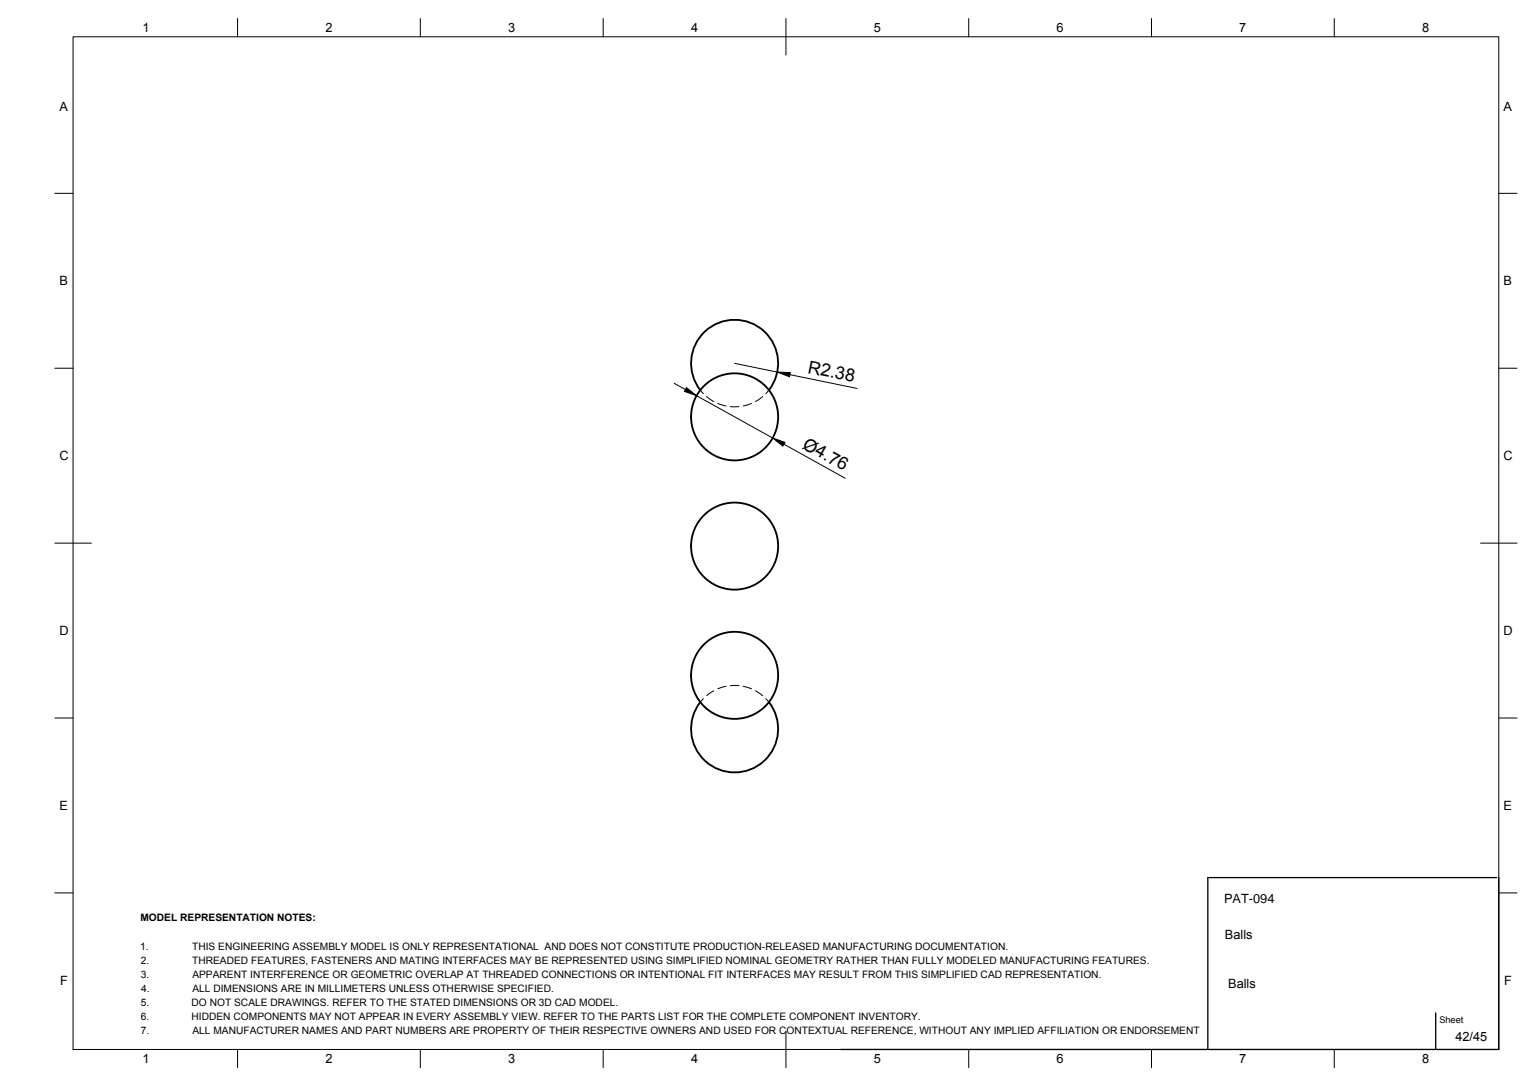
ISO-10303-21;
HEADER;
/* Generated by software containing ST-Developer
 * from STEP Tools, Inc. (www.steptools.com) 
 */

FILE_DESCRIPTION(
/* description */ ('Shaft runout checking stand'),
/* implementation_level */ '2;1');

FILE_NAME(
/* name */ 'Balls.step',
/* time_stamp */ '2026-11-02T21:12:33-08:00',
/* author */ (''),
/* organization */ (''),
/* preprocessor_version */ 'ST-DEVELOPER v20.2',
/* originating_system */ 'Autodesk Translation Framework v15.17.0.0',
/* authorisation */ '');

FILE_SCHEMA (('AUTOMOTIVE_DESIGN { 1 0 10303 214 3 1 1 }'));
ENDSEC;

DATA;
#10=MECHANICAL_DESIGN_GEOMETRIC_PRESENTATION_REPRESENTATION('',(#500,#501,#502,#503,#504,#505,#506,#507),#11748);
#11=SPHERICAL_SURFACE('',#7363,0.23815);
#12=SPHERICAL_SURFACE('',#7365,0.23815);
#13=SPHERICAL_SURFACE('',#7367,0.23815);
#14=SPHERICAL_SURFACE('',#7369,0.23815);
#15=SPHERICAL_SURFACE('',#7371,0.23815);
#16=SPHERICAL_SURFACE('',#7373,0.23815);
#17=SPHERICAL_SURFACE('',#7375,0.23815);
#18=SPHERICAL_SURFACE('',#7377,0.23815);
#414=SHAPE_REPRESENTATION_RELATIONSHIP('SRR','None',#11966,#457);
#457=ADVANCED_BREP_SHAPE_REPRESENTATION('',(#548,#549,#550,#551,#552,#553,
#554,#555),#11742);
#500=STYLED_ITEM('',(#12170),#548);
#501=STYLED_ITEM('',(#12170),#549);
#502=STYLED_ITEM('',(#12170),#550);
#503=STYLED_ITEM('',(#12170),#551);
#504=STYLED_ITEM('',(#12170),#552);
#505=STYLED_ITEM('',(#12170),#553);
#506=STYLED_ITEM('',(#12170),#554);
#507=STYLED_ITEM('',(#12170),#555);
#548=MANIFOLD_SOLID_BREP('Body1',#6246);
#549=MANIFOLD_SOLID_BREP('Body2',#6247);
#550=MANIFOLD_SOLID_BREP('Body3',#6248);
#551=MANIFOLD_SOLID_BREP('Body4',#6249);
#552=MANIFOLD_SOLID_BREP('Body5',#6250);
#553=MANIFOLD_SOLID_BREP('Body6',#6251);
#554=MANIFOLD_SOLID_BREP('Body7',#6252);
#555=MANIFOLD_SOLID_BREP('Body8',#6253);
#876=CIRCLE('',#7364,0.23815);
#877=CIRCLE('',#7366,0.23815);
#878=CIRCLE('',#7368,0.23815);
#879=CIRCLE('',#7370,0.23815);
#880=CIRCLE('',#7372,0.23815);
#881=CIRCLE('',#7374,0.23815);
#882=CIRCLE('',#7376,0.23815);
#883=CIRCLE('',#7378,0.23815);
#1359=FACE_OUTER_BOUND('',#1827,.T.);
#1360=FACE_OUTER_BOUND('',#1828,.T.);
#1361=FACE_OUTER_BOUND('',#1829,.T.);
#1362=FACE_OUTER_BOUND('',#1830,.T.);
#1363=FACE_OUTER_BOUND('',#1831,.T.);
#1364=FACE_OUTER_BOUND('',#1832,.T.);
#1365=FACE_OUTER_BOUND('',#1833,.T.);
#1366=FACE_OUTER_BOUND('',#1834,.T.);
#1827=EDGE_LOOP('',(#5420,#5421));
#1828=EDGE_LOOP('',(#5422,#5423));
#1829=EDGE_LOOP('',(#5424,#5425));
#1830=EDGE_LOOP('',(#5426,#5427));
#1831=EDGE_LOOP('',(#5428,#5429));
#1832=EDGE_LOOP('',(#5430,#5431));
#1833=EDGE_LOOP('',(#5432,#5433));
#1834=EDGE_LOOP('',(#5434,#5435));
#3258=VERTEX_POINT('',#11083);
#3259=VERTEX_POINT('',#11084);
#3260=VERTEX_POINT('',#11087);
#3261=VERTEX_POINT('',#11088);
#3262=VERTEX_POINT('',#11091);
#3263=VERTEX_POINT('',#11092);
#3264=VERTEX_POINT('',#11095);
#3265=VERTEX_POINT('',#11096);
#3266=VERTEX_POINT('',#11099);
#3267=VERTEX_POINT('',#11100);
#3268=VERTEX_POINT('',#11103);
#3269=VERTEX_POINT('',#11104);
#3270=VERTEX_POINT('',#11107);
#3271=VERTEX_POINT('',#11108);
#3272=VERTEX_POINT('',#11111);
#3273=VERTEX_POINT('',#11112);
#3996=EDGE_CURVE('',#3258,#3259,#876,.T.);
#3997=EDGE_CURVE('',#3260,#3261,#877,.T.);
#3998=EDGE_CURVE('',#3262,#3263,#878,.T.);
#3999=EDGE_CURVE('',#3264,#3265,#879,.T.);
#4000=EDGE_CURVE('',#3266,#3267,#880,.T.);
#4001=EDGE_CURVE('',#3268,#3269,#881,.T.);
#4002=EDGE_CURVE('',#3270,#3271,#882,.T.);
#4003=EDGE_CURVE('',#3272,#3273,#883,.T.);
#5420=ORIENTED_EDGE('',*,*,#3996,.T.);
#5421=ORIENTED_EDGE('',*,*,#3996,.F.);
#5422=ORIENTED_EDGE('',*,*,#3997,.T.);
#5423=ORIENTED_EDGE('',*,*,#3997,.F.);
#5424=ORIENTED_EDGE('',*,*,#3998,.T.);
#5425=ORIENTED_EDGE('',*,*,#3998,.F.);
#5426=ORIENTED_EDGE('',*,*,#3999,.T.);
#5427=ORIENTED_EDGE('',*,*,#3999,.F.);
#5428=ORIENTED_EDGE('',*,*,#4000,.T.);
#5429=ORIENTED_EDGE('',*,*,#4000,.F.);
#5430=ORIENTED_EDGE('',*,*,#4001,.T.);
#5431=ORIENTED_EDGE('',*,*,#4001,.F.);
#5432=ORIENTED_EDGE('',*,*,#4002,.T.);
#5433=ORIENTED_EDGE('',*,*,#4002,.F.);
#5434=ORIENTED_EDGE('',*,*,#4003,.T.);
#5435=ORIENTED_EDGE('',*,*,#4003,.F.);
#6159=ADVANCED_FACE('',(#1359),#11,.T.);
#6160=ADVANCED_FACE('',(#1360),#12,.T.);
#6161=ADVANCED_FACE('',(#1361),#13,.T.);
#6162=ADVANCED_FACE('',(#1362),#14,.T.);
#6163=ADVANCED_FACE('',(#1363),#15,.T.);
#6164=ADVANCED_FACE('',(#1364),#16,.T.);
#6165=ADVANCED_FACE('',(#1365),#17,.T.);
#6166=ADVANCED_FACE('',(#1366),#18,.T.);
#6246=CLOSED_SHELL('',(#6159));
#6247=CLOSED_SHELL('',(#6160));
#6248=CLOSED_SHELL('',(#6161));
#6249=CLOSED_SHELL('',(#6162));
#6250=CLOSED_SHELL('',(#6163));
#6251=CLOSED_SHELL('',(#6164));
#6252=CLOSED_SHELL('',(#6165));
#6253=CLOSED_SHELL('',(#6166));
#7362=AXIS2_PLACEMENT_3D('',#11081,#9203,#9204);
#7363=AXIS2_PLACEMENT_3D('',#11082,#9205,#9206);
#7364=AXIS2_PLACEMENT_3D('',#11085,#9207,#9208);
#7365=AXIS2_PLACEMENT_3D('',#11086,#9209,#9210);
#7366=AXIS2_PLACEMENT_3D('',#11089,#9211,#9212);
#7367=AXIS2_PLACEMENT_3D('',#11090,#9213,#9214);
#7368=AXIS2_PLACEMENT_3D('',#11093,#9215,#9216);
#7369=AXIS2_PLACEMENT_3D('',#11094,#9217,#9218);
#7370=AXIS2_PLACEMENT_3D('',#11097,#9219,#9220);
#7371=AXIS2_PLACEMENT_3D('',#11098,#9221,#9222);
#7372=AXIS2_PLACEMENT_3D('',#11101,#9223,#9224);
#7373=AXIS2_PLACEMENT_3D('',#11102,#9225,#9226);
#7374=AXIS2_PLACEMENT_3D('',#11105,#9227,#9228);
#7375=AXIS2_PLACEMENT_3D('',#11106,#9229,#9230);
#7376=AXIS2_PLACEMENT_3D('',#11109,#9231,#9232);
#7377=AXIS2_PLACEMENT_3D('',#11110,#9233,#9234);
#7378=AXIS2_PLACEMENT_3D('',#11113,#9235,#9236);
#9203=DIRECTION('axis',(0.,0.,1.));
#9204=DIRECTION('refdir',(1.,0.,0.));
#9205=DIRECTION('center_axis',(0.,0.,1.));
#9206=DIRECTION('ref_axis',(1.,0.,0.));
#9207=DIRECTION('center_axis',(1.22464679914735E-16,-1.,0.));
#9208=DIRECTION('ref_axis',(-1.,-1.22464679914735E-16,0.));
#9209=DIRECTION('center_axis',(0.707106781186548,0.,0.707106781186548));
#9210=DIRECTION('ref_axis',(0.707106781186548,0.,-0.707106781186548));
#9211=DIRECTION('center_axis',(8.65956056235494E-17,-1.,-8.65956056235493E-17));
#9212=DIRECTION('ref_axis',(-0.707106781186547,-1.22464679914735E-16,0.707106781186547));
#9213=DIRECTION('center_axis',(1.,0.,0.));
#9214=DIRECTION('ref_axis',(6.12323399573676E-17,0.,-1.));
#9215=DIRECTION('center_axis',(7.49879891330929E-33,-1.,-1.22464679914735E-16));
#9216=DIRECTION('ref_axis',(-6.12323399573676E-17,-1.22464679914735E-16,
1.));
#9217=DIRECTION('center_axis',(0.707106781186548,0.,-0.707106781186548));
#9218=DIRECTION('ref_axis',(-0.707106781186548,0.,-0.707106781186548));
#9219=DIRECTION('center_axis',(-8.65956056235493E-17,-1.,-8.65956056235494E-17));
#9220=DIRECTION('ref_axis',(0.707106781186547,-1.22464679914735E-16,0.707106781186547));
#9221=DIRECTION('center_axis',(0.,0.,-1.));
#9222=DIRECTION('ref_axis',(-1.,0.,-1.22464679914735E-16));
#9223=DIRECTION('center_axis',(-1.22464679914735E-16,-1.,-1.49975978266186E-32));
#9224=DIRECTION('ref_axis',(1.,-1.22464679914735E-16,1.22464679914735E-16));
#9225=DIRECTION('center_axis',(-0.707106781186547,0.,-0.707106781186548));
#9226=DIRECTION('ref_axis',(-0.707106781186548,0.,0.707106781186547));
#9227=DIRECTION('center_axis',(-8.65956056235493E-17,-1.,8.65956056235493E-17));
#9228=DIRECTION('ref_axis',(0.707106781186548,-1.22464679914735E-16,-0.707106781186547));
#9229=DIRECTION('center_axis',(-1.,0.,0.));
#9230=DIRECTION('ref_axis',(-1.83697019872103E-16,0.,1.));
#9231=DIRECTION('center_axis',(-2.24963967399279E-32,-1.,1.22464679914735E-16));
#9232=DIRECTION('ref_axis',(1.83697019872103E-16,-1.22464679914735E-16,
-1.));
#9233=DIRECTION('center_axis',(-0.707106781186548,0.,0.707106781186548));
#9234=DIRECTION('ref_axis',(0.707106781186547,0.,0.707106781186548));
#9235=DIRECTION('center_axis',(8.65956056235493E-17,-1.,8.65956056235493E-17));
#9236=DIRECTION('ref_axis',(-0.707106781186547,-1.22464679914735E-16,-0.707106781186548));
#11081=CARTESIAN_POINT('',(0.,0.,0.));
#11082=CARTESIAN_POINT('Origin',(1.,0.,0.));
#11083=CARTESIAN_POINT('',(1.,-1.78583896120461E-33,0.23815));
#11084=CARTESIAN_POINT('',(1.,-1.78583896120461E-33,-0.23815));
#11085=CARTESIAN_POINT('Origin',(1.,0.,0.));
#11086=CARTESIAN_POINT('Origin',(0.707106781186548,0.,-0.707106781186547));
#11087=CARTESIAN_POINT('',(0.875504261126124,-1.78583896120461E-33,-0.538709301246971));
#11088=CARTESIAN_POINT('',(0.538709301246971,-1.78583896120461E-33,-0.875504261126124));
#11089=CARTESIAN_POINT('Origin',(0.707106781186548,0.,-0.707106781186547));
#11090=CARTESIAN_POINT('Origin',(6.12323399573677E-17,0.,-1.));
#11091=CARTESIAN_POINT('',(0.23815,-1.78583896120461E-33,-1.));
#11092=CARTESIAN_POINT('',(-0.23815,-1.78583896120461E-33,-1.));
#11093=CARTESIAN_POINT('Origin',(6.12323399573677E-17,0.,-1.));
#11094=CARTESIAN_POINT('Origin',(-0.707106781186547,0.,-0.707106781186548));
#11095=CARTESIAN_POINT('',(-0.538709301246971,-1.78583896120461E-33,-0.875504261126124));
#11096=CARTESIAN_POINT('',(-0.875504261126124,-1.78583896120461E-33,-0.538709301246971));
#11097=CARTESIAN_POINT('Origin',(-0.707106781186547,0.,-0.707106781186548));
#11098=CARTESIAN_POINT('Origin',(-1.,0.,-1.22464679914735E-16));
#11099=CARTESIAN_POINT('',(-1.,-1.78583896120461E-33,-0.23815));
#11100=CARTESIAN_POINT('',(-1.,-1.78583896120461E-33,0.23815));
#11101=CARTESIAN_POINT('Origin',(-1.,0.,-1.22464679914735E-16));
#11102=CARTESIAN_POINT('Origin',(-0.707106781186548,0.,0.707106781186547));
#11103=CARTESIAN_POINT('',(-0.875504261126124,-7.94881478324376E-33,0.538709301246971));
#11104=CARTESIAN_POINT('',(-0.538709301246971,4.37713686083455E-33,0.875504261126124));
#11105=CARTESIAN_POINT('Origin',(-0.707106781186548,0.,0.707106781186547));
#11106=CARTESIAN_POINT('Origin',(-1.83697019872103E-16,0.,1.));
#11107=CARTESIAN_POINT('',(-0.23815,-1.78583896120461E-33,1.));
#11108=CARTESIAN_POINT('',(0.23815,-1.78583896120461E-33,1.));
#11109=CARTESIAN_POINT('Origin',(-1.83697019872103E-16,0.,1.));
#11110=CARTESIAN_POINT('Origin',(0.707106781186547,0.,0.707106781186548));
#11111=CARTESIAN_POINT('',(0.538709301246971,-4.86732687222419E-33,0.875504261126124));
#11112=CARTESIAN_POINT('',(0.875504261126124,1.29564894981497E-33,0.538709301246971));
#11113=CARTESIAN_POINT('Origin',(0.707106781186547,0.,0.707106781186548));
#11693=UNCERTAINTY_MEASURE_WITH_UNIT(LENGTH_MEASURE(0.001),#11749,
'DISTANCE_ACCURACY_VALUE',
'Maximum model space distance between geometric entities at asserted c
onnectivities');
#11699=UNCERTAINTY_MEASURE_WITH_UNIT(LENGTH_MEASURE(0.001),#11749,
'DISTANCE_ACCURACY_VALUE',
'Maximum model space distance between geometric entities at asserted c
onnectivities');
#11742=(
GEOMETRIC_REPRESENTATION_CONTEXT(3)
GLOBAL_UNCERTAINTY_ASSIGNED_CONTEXT((#11693))
GLOBAL_UNIT_ASSIGNED_CONTEXT((#11749,#11751,#11752))
REPRESENTATION_CONTEXT('','3D')
);
#11748=(
GEOMETRIC_REPRESENTATION_CONTEXT(3)
GLOBAL_UNCERTAINTY_ASSIGNED_CONTEXT((#11699))
GLOBAL_UNIT_ASSIGNED_CONTEXT((#11749,#11751,#11752))
REPRESENTATION_CONTEXT('','3D')
);
#11749=(
LENGTH_UNIT()
NAMED_UNIT(*)
SI_UNIT(.CENTI.,.METRE.)
);
#11751=(
NAMED_UNIT(*)
PLANE_ANGLE_UNIT()
SI_UNIT($,.RADIAN.)
);
#11752=(
NAMED_UNIT(*)
SI_UNIT($,.STERADIAN.)
SOLID_ANGLE_UNIT()
);
#11795=SHAPE_DEFINITION_REPRESENTATION(#11903,#11966);
#11903=PRODUCT_DEFINITION_SHAPE('',$,#12015);
#11966=SHAPE_REPRESENTATION('',(#7362),#11742);
#11972=PRODUCT_DEFINITION_CONTEXT('part definition',#12118,'design');
#12015=PRODUCT_DEFINITION('Balls','Balls',#12063,#11972);
#12063=PRODUCT_DEFINITION_FORMATION('',$,#12162);
#12118=APPLICATION_CONTEXT(
'Core Data for Automotive Mechanical Design Process');
#12119=PRODUCT_CONTEXT('part definition',#12118,'mechanical');
#12162=PRODUCT('Balls','Balls','Balls',(#12119));
#12170=PRESENTATION_STYLE_ASSIGNMENT((#12175));
#12175=SURFACE_STYLE_USAGE(.BOTH.,#12180);
#12180=SURFACE_SIDE_STYLE('',(#12185));
#12185=SURFACE_STYLE_FILL_AREA(#12190);
#12190=FILL_AREA_STYLE('CAD Library Painted - Steel gray',(#12195));
#12195=FILL_AREA_STYLE_COLOUR('CAD Library Painted - Steel gray',#12200);
#12200=COLOUR_RGB('CAD Library Painted - Steel gray',0.592156862745098,
0.631372549019608,0.67843137254902);
ENDSEC;
END-ISO-10303-21;
